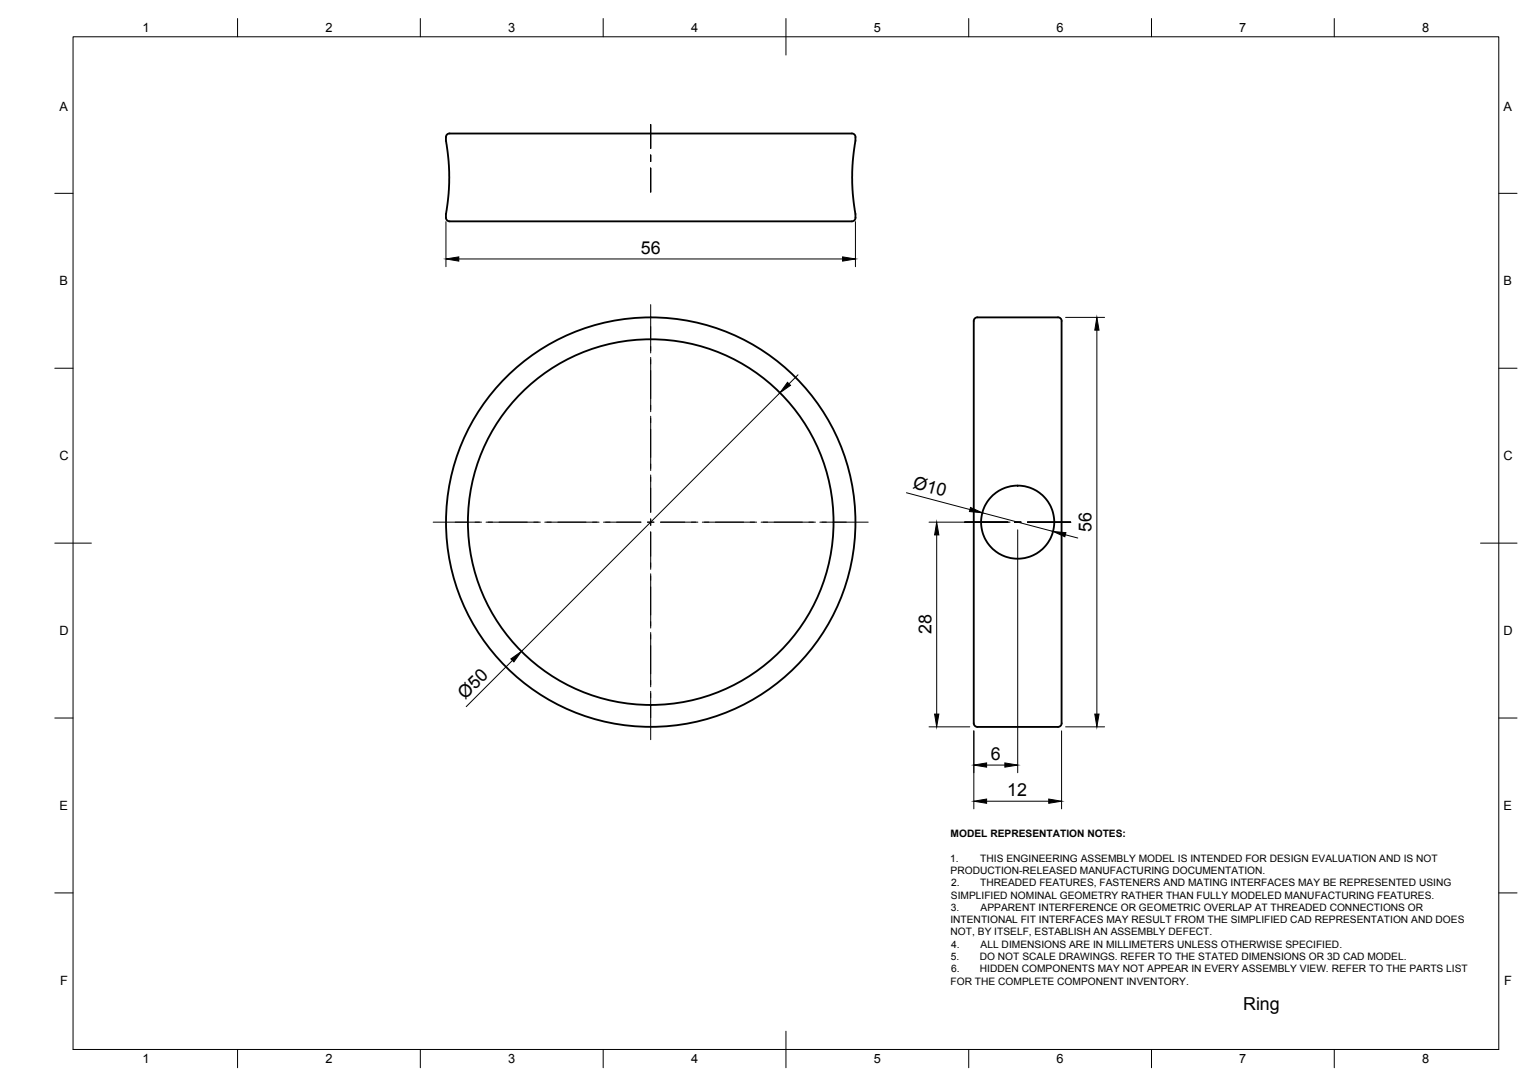
ISO-10303-21;
HEADER;
/* Generated by software containing ST-Developer
 * from STEP Tools, Inc. (www.steptools.com) 
 */

FILE_DESCRIPTION(
/* description */ (''),
/* implementation_level */ '2;1');

FILE_NAME(
/* name */ 'Ring.step',
/* time_stamp */ '2026-10-06T12:52:28-07:00',
/* author */ (''),
/* organization */ (''),
/* preprocessor_version */ 'ST-DEVELOPER v20.2',
/* originating_system */ 'Autodesk Translation Framework v15.15.0.0',
/* authorisation */ '');

FILE_SCHEMA (('AUTOMOTIVE_DESIGN { 1 0 10303 214 3 1 1 }'));
ENDSEC;

DATA;
#10=MECHANICAL_DESIGN_GEOMETRIC_PRESENTATION_REPRESENTATION('',(#73),#34403);
#57=SHAPE_REPRESENTATION_RELATIONSHIP('SRR','None',#34435,#65);
#65=ADVANCED_BREP_SHAPE_REPRESENTATION('',(#81),#34395);
#73=STYLED_ITEM('',(#34484),#81);
#81=MANIFOLD_SOLID_BREP('Body1',#4382);
#89=FACE_BOUND('',#751,.T.);
#90=FACE_BOUND('',#753,.T.);
#91=FACE_BOUND('',#754,.T.);
#92=FACE_BOUND('',#757,.T.);
#93=FACE_BOUND('',#758,.T.);
#94=FACE_BOUND('',#761,.T.);
#125=PLANE('',#4488);
#126=PLANE('',#4503);
#160=CIRCLE('',#4484,25.5);
#161=CIRCLE('',#4485,0.5);
#162=CIRCLE('',#4486,25.);
#163=CIRCLE('',#4487,25.);
#164=CIRCLE('',#4489,27.5);
#165=CIRCLE('',#4491,25.);
#166=CIRCLE('',#4492,25.);
#167=CIRCLE('',#4494,0.5);
#168=CIRCLE('',#4495,28.);
#169=CIRCLE('',#4496,28.);
#170=CIRCLE('',#4498,28.);
#171=CIRCLE('',#4499,28.);
#172=CIRCLE('',#4501,27.5);
#173=CIRCLE('',#4502,0.5);
#174=CIRCLE('',#4504,25.5);
#175=CIRCLE('',#4506,0.5);
#446=TOROIDAL_SURFACE('',#4483,25.5,0.5);
#447=TOROIDAL_SURFACE('',#4493,27.5,0.5);
#448=TOROIDAL_SURFACE('',#4500,27.5,0.5);
#449=TOROIDAL_SURFACE('',#4505,25.5,0.5);
#516=FACE_OUTER_BOUND('',#747,.T.);
#517=FACE_OUTER_BOUND('',#748,.T.);
#518=FACE_OUTER_BOUND('',#749,.T.);
#519=FACE_OUTER_BOUND('',#750,.T.);
#520=FACE_OUTER_BOUND('',#752,.T.);
#521=FACE_OUTER_BOUND('',#755,.T.);
#522=FACE_OUTER_BOUND('',#756,.T.);
#523=FACE_OUTER_BOUND('',#759,.T.);
#524=FACE_OUTER_BOUND('',#760,.T.);
#525=FACE_OUTER_BOUND('',#762,.T.);
#747=EDGE_LOOP('',(#2683,#2684,#2685,#2686,#2687,#2688));
#748=EDGE_LOOP('',(#2689,#2690,#2691,#2692,#2693,#2694));
#749=EDGE_LOOP('',(#2695,#2696,#2697,#2698,#2699));
#750=EDGE_LOOP('',(#2700));
#751=EDGE_LOOP('',(#2701));
#752=EDGE_LOOP('',(#2702,#2703,#2704,#2705,#2706,#2707));
#753=EDGE_LOOP('',(#2708,#2709));
#754=EDGE_LOOP('',(#2710,#2711));
#755=EDGE_LOOP('',(#2712,#2713,#2714,#2715,#2716));
#756=EDGE_LOOP('',(#2717,#2718,#2719,#2720,#2721,#2722));
#757=EDGE_LOOP('',(#2723,#2724));
#758=EDGE_LOOP('',(#2725,#2726));
#759=EDGE_LOOP('',(#2727,#2728,#2729,#2730,#2731));
#760=EDGE_LOOP('',(#2732));
#761=EDGE_LOOP('',(#2733));
#762=EDGE_LOOP('',(#2734,#2735,#2736,#2737,#2738));
#1014=LINE('',#6230,#1151);
#1015=LINE('',#6308,#1152);
#1016=LINE('',#6362,#1153);
#1017=LINE('',#6371,#1154);
#1151=VECTOR('',#5009,5.);
#1152=VECTOR('',#5012,5.);
#1153=VECTOR('',#5033,25.);
#1154=VECTOR('',#5044,28.);
#1288=B_SPLINE_CURVE_WITH_KNOTS('',3,(#6193,#6194,#6195,#6196,#6197,#6198,
#6199,#6200,#6201,#6202,#6203,#6204,#6205,#6206,#6207,#6208,#6209,#6210),
 .UNSPECIFIED.,.F.,.F.,(4,2,2,2,2,2,2,2,4),(0.,0.188782577961406,0.377565155922812,
0.566341063168598,0.755116970414385,0.94389287766017,1.13266878490596,1.32145136286736,
1.51023394082877),.UNSPECIFIED.);
#1289=B_SPLINE_CURVE_WITH_KNOTS('',3,(#6211,#6212,#6213,#6214,#6215,#6216,
#6217,#6218,#6219,#6220,#6221,#6222,#6223,#6224,#6225,#6226,#6227,#6228),
 .UNSPECIFIED.,.F.,.F.,(4,2,2,2,2,2,2,2,4),(1.51023394082877,1.69901651879018,
1.88779909675158,2.07657500399737,2.26535091124315,2.45412681848894,2.64290272573473,
2.83168530369613,3.02046788165754),.UNSPECIFIED.);
#1290=B_SPLINE_CURVE_WITH_KNOTS('',3,(#6232,#6233,#6234,#6235,#6236,#6237,
#6238,#6239,#6240,#6241,#6242,#6243,#6244,#6245,#6246,#6247,#6248,#6249),
 .UNSPECIFIED.,.F.,.F.,(4,2,2,2,2,2,2,2,4),(-3.02227736861757,-2.83337974067247,
-2.64448211272738,-2.45559506959528,-2.26670802646318,-2.07782098333108,
-1.88893394019898,-1.70003631225388,-1.51113868430879),.UNSPECIFIED.);
#1291=B_SPLINE_CURVE_WITH_KNOTS('',3,(#6250,#6251,#6252,#6253,#6254,#6255,
#6256,#6257,#6258,#6259,#6260,#6261,#6262,#6263,#6264,#6265,#6266,#6267),
 .UNSPECIFIED.,.F.,.F.,(4,2,2,2,2,2,2,2,4),(-1.51113868430879,-1.32224105636369,
-1.13334342841859,-0.944456385286492,-0.755569342154393,-0.566682299022294,
-0.377795255890194,-0.188897627945097,0.),.UNSPECIFIED.);
#1292=B_SPLINE_CURVE_WITH_KNOTS('',3,(#6271,#6272,#6273,#6274,#6275,#6276,
#6277,#6278,#6279,#6280,#6281,#6282,#6283,#6284,#6285,#6286,#6287,#6288),
 .UNSPECIFIED.,.F.,.F.,(4,2,2,2,2,2,2,2,4),(-3.02227736861757,-2.83337974067247,
-2.64448211272738,-2.45559506959528,-2.26670802646318,-2.07782098333108,
-1.88893394019898,-1.70003631225388,-1.51113868430879),.UNSPECIFIED.);
#1293=B_SPLINE_CURVE_WITH_KNOTS('',3,(#6289,#6290,#6291,#6292,#6293,#6294,
#6295,#6296,#6297,#6298,#6299,#6300,#6301,#6302,#6303,#6304,#6305,#6306),
 .UNSPECIFIED.,.F.,.F.,(4,2,2,2,2,2,2,2,4),(-1.51113868430879,-1.32224105636369,
-1.13334342841859,-0.944456385286492,-0.755569342154393,-0.566682299022294,
-0.377795255890194,-0.188897627945097,0.),.UNSPECIFIED.);
#1294=B_SPLINE_CURVE_WITH_KNOTS('',3,(#6310,#6311,#6312,#6313,#6314,#6315,
#6316,#6317,#6318,#6319,#6320,#6321,#6322,#6323,#6324,#6325,#6326,#6327),
 .UNSPECIFIED.,.F.,.F.,(4,2,2,2,2,2,2,2,4),(0.,0.188782577961406,0.377565155922812,
0.566341063168599,0.755116970414385,0.943892877660171,1.13266878490596,
1.32145136286736,1.51023394082877),.UNSPECIFIED.);
#1295=B_SPLINE_CURVE_WITH_KNOTS('',3,(#6328,#6329,#6330,#6331,#6332,#6333,
#6334,#6335,#6336,#6337,#6338,#6339,#6340,#6341,#6342,#6343,#6344,#6345),
 .UNSPECIFIED.,.F.,.F.,(4,2,2,2,2,2,2,2,4),(1.51023394082877,1.69901651879018,
1.88779909675158,2.07657500399737,2.26535091124315,2.45412681848894,2.64290272573473,
2.83168530369613,3.02046788165754),.UNSPECIFIED.);
#1540=VERTEX_POINT('',#6191);
#1541=VERTEX_POINT('',#6192);
#1542=VERTEX_POINT('',#6229);
#1543=VERTEX_POINT('',#6231);
#1544=VERTEX_POINT('',#6269);
#1545=VERTEX_POINT('',#6270);
#1546=VERTEX_POINT('',#6307);
#1547=VERTEX_POINT('',#6309);
#1548=VERTEX_POINT('',#6347);
#1549=VERTEX_POINT('',#6349);
#1550=VERTEX_POINT('',#6351);
#1551=VERTEX_POINT('',#6355);
#1552=VERTEX_POINT('',#6358);
#1553=VERTEX_POINT('',#6359);
#1554=VERTEX_POINT('',#6364);
#1555=VERTEX_POINT('',#6366);
#1556=VERTEX_POINT('',#6370);
#1557=VERTEX_POINT('',#6372);
#1558=VERTEX_POINT('',#6376);
#1559=VERTEX_POINT('',#6380);
#2006=EDGE_CURVE('',#1540,#1541,#1288,.T.);
#2007=EDGE_CURVE('',#1541,#1540,#1289,.T.);
#2008=EDGE_CURVE('',#1541,#1542,#1014,.T.);
#2009=EDGE_CURVE('',#1543,#1542,#1290,.T.);
#2010=EDGE_CURVE('',#1542,#1543,#1291,.T.);
#2011=EDGE_CURVE('',#1544,#1545,#1292,.T.);
#2012=EDGE_CURVE('',#1545,#1544,#1293,.T.);
#2013=EDGE_CURVE('',#1545,#1546,#1015,.T.);
#2014=EDGE_CURVE('',#1547,#1546,#1294,.T.);
#2015=EDGE_CURVE('',#1546,#1547,#1295,.T.);
#2016=EDGE_CURVE('',#1548,#1548,#160,.T.);
#2017=EDGE_CURVE('',#1548,#1549,#161,.T.);
#2018=EDGE_CURVE('',#1549,#1550,#162,.T.);
#2019=EDGE_CURVE('',#1550,#1549,#163,.T.);
#2020=EDGE_CURVE('',#1551,#1551,#164,.T.);
#2021=EDGE_CURVE('',#1552,#1553,#165,.T.);
#2022=EDGE_CURVE('',#1553,#1552,#166,.T.);
#2023=EDGE_CURVE('',#1553,#1550,#1016,.T.);
#2024=EDGE_CURVE('',#1551,#1554,#167,.T.);
#2025=EDGE_CURVE('',#1554,#1555,#168,.T.);
#2026=EDGE_CURVE('',#1555,#1554,#169,.T.);
#2027=EDGE_CURVE('',#1555,#1556,#1017,.T.);
#2028=EDGE_CURVE('',#1557,#1556,#170,.T.);
#2029=EDGE_CURVE('',#1556,#1557,#171,.T.);
#2030=EDGE_CURVE('',#1558,#1558,#172,.T.);
#2031=EDGE_CURVE('',#1558,#1557,#173,.T.);
#2032=EDGE_CURVE('',#1559,#1559,#174,.T.);
#2033=EDGE_CURVE('',#1559,#1552,#175,.T.);
#2683=ORIENTED_EDGE('',*,*,#2006,.F.);
#2684=ORIENTED_EDGE('',*,*,#2007,.F.);
#2685=ORIENTED_EDGE('',*,*,#2008,.T.);
#2686=ORIENTED_EDGE('',*,*,#2009,.F.);
#2687=ORIENTED_EDGE('',*,*,#2010,.F.);
#2688=ORIENTED_EDGE('',*,*,#2008,.F.);
#2689=ORIENTED_EDGE('',*,*,#2011,.F.);
#2690=ORIENTED_EDGE('',*,*,#2012,.F.);
#2691=ORIENTED_EDGE('',*,*,#2013,.T.);
#2692=ORIENTED_EDGE('',*,*,#2014,.F.);
#2693=ORIENTED_EDGE('',*,*,#2015,.F.);
#2694=ORIENTED_EDGE('',*,*,#2013,.F.);
#2695=ORIENTED_EDGE('',*,*,#2016,.T.);
#2696=ORIENTED_EDGE('',*,*,#2017,.T.);
#2697=ORIENTED_EDGE('',*,*,#2018,.T.);
#2698=ORIENTED_EDGE('',*,*,#2019,.T.);
#2699=ORIENTED_EDGE('',*,*,#2017,.F.);
#2700=ORIENTED_EDGE('',*,*,#2020,.F.);
#2701=ORIENTED_EDGE('',*,*,#2016,.F.);
#2702=ORIENTED_EDGE('',*,*,#2021,.F.);
#2703=ORIENTED_EDGE('',*,*,#2022,.F.);
#2704=ORIENTED_EDGE('',*,*,#2023,.T.);
#2705=ORIENTED_EDGE('',*,*,#2018,.F.);
#2706=ORIENTED_EDGE('',*,*,#2019,.F.);
#2707=ORIENTED_EDGE('',*,*,#2023,.F.);
#2708=ORIENTED_EDGE('',*,*,#2011,.T.);
#2709=ORIENTED_EDGE('',*,*,#2012,.T.);
#2710=ORIENTED_EDGE('',*,*,#2009,.T.);
#2711=ORIENTED_EDGE('',*,*,#2010,.T.);
#2712=ORIENTED_EDGE('',*,*,#2020,.T.);
#2713=ORIENTED_EDGE('',*,*,#2024,.T.);
#2714=ORIENTED_EDGE('',*,*,#2025,.T.);
#2715=ORIENTED_EDGE('',*,*,#2026,.T.);
#2716=ORIENTED_EDGE('',*,*,#2024,.F.);
#2717=ORIENTED_EDGE('',*,*,#2026,.F.);
#2718=ORIENTED_EDGE('',*,*,#2027,.T.);
#2719=ORIENTED_EDGE('',*,*,#2028,.F.);
#2720=ORIENTED_EDGE('',*,*,#2029,.F.);
#2721=ORIENTED_EDGE('',*,*,#2027,.F.);
#2722=ORIENTED_EDGE('',*,*,#2025,.F.);
#2723=ORIENTED_EDGE('',*,*,#2014,.T.);
#2724=ORIENTED_EDGE('',*,*,#2015,.T.);
#2725=ORIENTED_EDGE('',*,*,#2006,.T.);
#2726=ORIENTED_EDGE('',*,*,#2007,.T.);
#2727=ORIENTED_EDGE('',*,*,#2030,.T.);
#2728=ORIENTED_EDGE('',*,*,#2031,.T.);
#2729=ORIENTED_EDGE('',*,*,#2028,.T.);
#2730=ORIENTED_EDGE('',*,*,#2029,.T.);
#2731=ORIENTED_EDGE('',*,*,#2031,.F.);
#2732=ORIENTED_EDGE('',*,*,#2030,.F.);
#2733=ORIENTED_EDGE('',*,*,#2032,.F.);
#2734=ORIENTED_EDGE('',*,*,#2032,.T.);
#2735=ORIENTED_EDGE('',*,*,#2033,.T.);
#2736=ORIENTED_EDGE('',*,*,#2021,.T.);
#2737=ORIENTED_EDGE('',*,*,#2022,.T.);
#2738=ORIENTED_EDGE('',*,*,#2033,.F.);
#4037=CYLINDRICAL_SURFACE('',#4481,5.);
#4038=CYLINDRICAL_SURFACE('',#4482,5.);
#4039=CYLINDRICAL_SURFACE('',#4490,25.);
#4040=CYLINDRICAL_SURFACE('',#4497,28.);
#4151=ADVANCED_FACE('',(#516),#4037,.F.);
#4152=ADVANCED_FACE('',(#517),#4038,.F.);
#4153=ADVANCED_FACE('',(#518),#446,.T.);
#4154=ADVANCED_FACE('',(#519,#89),#125,.T.);
#4155=ADVANCED_FACE('',(#520,#90,#91),#4039,.F.);
#4156=ADVANCED_FACE('',(#521),#447,.T.);
#4157=ADVANCED_FACE('',(#522,#92,#93),#4040,.T.);
#4158=ADVANCED_FACE('',(#523),#448,.T.);
#4159=ADVANCED_FACE('',(#524,#94),#126,.F.);
#4160=ADVANCED_FACE('',(#525),#449,.T.);
#4382=CLOSED_SHELL('',(#4151,#4152,#4153,#4154,#4155,#4156,#4157,#4158,
#4159,#4160));
#4480=AXIS2_PLACEMENT_3D('',#6189,#5005,#5006);
#4481=AXIS2_PLACEMENT_3D('',#6190,#5007,#5008);
#4482=AXIS2_PLACEMENT_3D('',#6268,#5010,#5011);
#4483=AXIS2_PLACEMENT_3D('',#6346,#5013,#5014);
#4484=AXIS2_PLACEMENT_3D('',#6348,#5015,#5016);
#4485=AXIS2_PLACEMENT_3D('',#6350,#5017,#5018);
#4486=AXIS2_PLACEMENT_3D('',#6352,#5019,#5020);
#4487=AXIS2_PLACEMENT_3D('',#6353,#5021,#5022);
#4488=AXIS2_PLACEMENT_3D('',#6354,#5023,#5024);
#4489=AXIS2_PLACEMENT_3D('',#6356,#5025,#5026);
#4490=AXIS2_PLACEMENT_3D('',#6357,#5027,#5028);
#4491=AXIS2_PLACEMENT_3D('',#6360,#5029,#5030);
#4492=AXIS2_PLACEMENT_3D('',#6361,#5031,#5032);
#4493=AXIS2_PLACEMENT_3D('',#6363,#5034,#5035);
#4494=AXIS2_PLACEMENT_3D('',#6365,#5036,#5037);
#4495=AXIS2_PLACEMENT_3D('',#6367,#5038,#5039);
#4496=AXIS2_PLACEMENT_3D('',#6368,#5040,#5041);
#4497=AXIS2_PLACEMENT_3D('',#6369,#5042,#5043);
#4498=AXIS2_PLACEMENT_3D('',#6373,#5045,#5046);
#4499=AXIS2_PLACEMENT_3D('',#6374,#5047,#5048);
#4500=AXIS2_PLACEMENT_3D('',#6375,#5049,#5050);
#4501=AXIS2_PLACEMENT_3D('',#6377,#5051,#5052);
#4502=AXIS2_PLACEMENT_3D('',#6378,#5053,#5054);
#4503=AXIS2_PLACEMENT_3D('',#6379,#5055,#5056);
#4504=AXIS2_PLACEMENT_3D('',#6381,#5057,#5058);
#4505=AXIS2_PLACEMENT_3D('',#6382,#5059,#5060);
#4506=AXIS2_PLACEMENT_3D('',#6383,#5061,#5062);
#5005=DIRECTION('axis',(0.,0.,1.));
#5006=DIRECTION('refdir',(1.,0.,0.));
#5007=DIRECTION('center_axis',(0.,0.,1.));
#5008=DIRECTION('ref_axis',(1.,0.,0.));
#5009=DIRECTION('',(0.,0.,1.));
#5010=DIRECTION('center_axis',(0.,0.,1.));
#5011=DIRECTION('ref_axis',(1.,0.,0.));
#5012=DIRECTION('',(0.,0.,1.));
#5013=DIRECTION('center_axis',(0.,-1.,0.));
#5014=DIRECTION('ref_axis',(0.,0.,-1.));
#5015=DIRECTION('center_axis',(0.,1.,0.));
#5016=DIRECTION('ref_axis',(1.,0.,0.));
#5017=DIRECTION('center_axis',(-1.,0.,-1.22464679914735E-16));
#5018=DIRECTION('ref_axis',(-1.22464679914735E-16,0.,1.));
#5019=DIRECTION('center_axis',(0.,-1.,0.));
#5020=DIRECTION('ref_axis',(1.,0.,0.));
#5021=DIRECTION('center_axis',(0.,-1.,0.));
#5022=DIRECTION('ref_axis',(1.,0.,0.));
#5023=DIRECTION('center_axis',(0.,1.,0.));
#5024=DIRECTION('ref_axis',(1.,0.,0.));
#5025=DIRECTION('center_axis',(0.,-1.,0.));
#5026=DIRECTION('ref_axis',(1.,0.,0.));
#5027=DIRECTION('center_axis',(0.,1.,0.));
#5028=DIRECTION('ref_axis',(1.,0.,0.));
#5029=DIRECTION('center_axis',(0.,1.,0.));
#5030=DIRECTION('ref_axis',(1.,0.,0.));
#5031=DIRECTION('center_axis',(0.,1.,0.));
#5032=DIRECTION('ref_axis',(1.,0.,0.));
#5033=DIRECTION('',(0.,1.,0.));
#5034=DIRECTION('center_axis',(0.,1.,0.));
#5035=DIRECTION('ref_axis',(0.,0.,1.));
#5036=DIRECTION('center_axis',(-1.,0.,1.22464679914735E-16));
#5037=DIRECTION('ref_axis',(-1.22464679914735E-16,0.,-1.));
#5038=DIRECTION('center_axis',(0.,1.,0.));
#5039=DIRECTION('ref_axis',(1.,0.,0.));
#5040=DIRECTION('center_axis',(0.,1.,0.));
#5041=DIRECTION('ref_axis',(1.,0.,0.));
#5042=DIRECTION('center_axis',(0.,1.,0.));
#5043=DIRECTION('ref_axis',(1.,0.,0.));
#5044=DIRECTION('',(0.,-1.,0.));
#5045=DIRECTION('center_axis',(0.,-1.,0.));
#5046=DIRECTION('ref_axis',(1.,0.,0.));
#5047=DIRECTION('center_axis',(0.,-1.,0.));
#5048=DIRECTION('ref_axis',(1.,0.,0.));
#5049=DIRECTION('center_axis',(0.,-1.,0.));
#5050=DIRECTION('ref_axis',(0.,0.,-1.));
#5051=DIRECTION('center_axis',(0.,1.,0.));
#5052=DIRECTION('ref_axis',(1.,0.,0.));
#5053=DIRECTION('center_axis',(-1.,0.,-1.22464679914735E-16));
#5054=DIRECTION('ref_axis',(-1.22464679914735E-16,0.,1.));
#5055=DIRECTION('center_axis',(0.,1.,0.));
#5056=DIRECTION('ref_axis',(1.,0.,0.));
#5057=DIRECTION('center_axis',(0.,-1.,0.));
#5058=DIRECTION('ref_axis',(1.,0.,0.));
#5059=DIRECTION('center_axis',(0.,1.,0.));
#5060=DIRECTION('ref_axis',(0.,0.,1.));
#5061=DIRECTION('center_axis',(-1.,0.,1.22464679914735E-16));
#5062=DIRECTION('ref_axis',(-1.22464679914735E-16,0.,-1.));
#6189=CARTESIAN_POINT('',(0.,0.,0.));
#6190=CARTESIAN_POINT('Origin',(0.,0.,0.));
#6191=CARTESIAN_POINT('',(5.,0.,-27.5499546279118));
#6192=CARTESIAN_POINT('',(-5.,-3.06161699786838E-16,-27.5499546279118));
#6193=CARTESIAN_POINT('Ctrl Pts',(5.,1.38777878078145E-16,-27.5499546279118));
#6194=CARTESIAN_POINT('Ctrl Pts',(5.,0.629275259871354,-27.5499546279118));
#6195=CARTESIAN_POINT('Ctrl Pts',(4.87396226264421,1.29954919562912,-27.5737468441049));
#6196=CARTESIAN_POINT('Ctrl Pts',(4.36328000904425,2.53103238085929,-27.6591541770631));
#6197=CARTESIAN_POINT('Ctrl Pts',(3.97870723422023,3.09236057764524,-27.7194782327905));
#6198=CARTESIAN_POINT('Ctrl Pts',(3.09237623737018,3.9786915744953,-27.832297423241));
#6199=CARTESIAN_POINT('Ctrl Pts',(2.53104134263485,4.3632766282051,-27.8921989820475));
#6200=CARTESIAN_POINT('Ctrl Pts',(1.29953505458189,4.87396779126795,-27.9766356618315));
#6201=CARTESIAN_POINT('Ctrl Pts',(0.62925302415262,5.,-28.));
#6202=CARTESIAN_POINT('Ctrl Pts',(-0.62925302415262,5.,-28.));
#6203=CARTESIAN_POINT('Ctrl Pts',(-1.29953505458189,4.87396779126795,-27.9766356618315));
#6204=CARTESIAN_POINT('Ctrl Pts',(-2.53104134263485,4.3632766282051,-27.8921989820475));
#6205=CARTESIAN_POINT('Ctrl Pts',(-3.09237623737018,3.9786915744953,-27.832297423241));
#6206=CARTESIAN_POINT('Ctrl Pts',(-3.97870723422023,3.09236057764524,-27.7194782327905));
#6207=CARTESIAN_POINT('Ctrl Pts',(-4.36328000904425,2.53103238085929,-27.6591541770631));
#6208=CARTESIAN_POINT('Ctrl Pts',(-4.87396226264421,1.29954919562912,-27.5737468441049));
#6209=CARTESIAN_POINT('Ctrl Pts',(-5.,0.629275259871354,-27.5499546279118));
#6210=CARTESIAN_POINT('Ctrl Pts',(-5.,-1.38777878078145E-16,-27.5499546279118));
#6211=CARTESIAN_POINT('Ctrl Pts',(-5.,0.,-27.5499546279118));
#6212=CARTESIAN_POINT('Ctrl Pts',(-5.,-0.629275259871354,-27.5499546279118));
#6213=CARTESIAN_POINT('Ctrl Pts',(-4.87396226264421,-1.29954919562912,-27.5737468441049));
#6214=CARTESIAN_POINT('Ctrl Pts',(-4.36328000904425,-2.53103238085929,-27.6591541770631));
#6215=CARTESIAN_POINT('Ctrl Pts',(-3.97870723422023,-3.09236057764524,-27.7194782327905));
#6216=CARTESIAN_POINT('Ctrl Pts',(-3.09237623737018,-3.9786915744953,-27.832297423241));
#6217=CARTESIAN_POINT('Ctrl Pts',(-2.53104134263485,-4.3632766282051,-27.8921989820475));
#6218=CARTESIAN_POINT('Ctrl Pts',(-1.29953505458189,-4.87396779126795,-27.9766356618315));
#6219=CARTESIAN_POINT('Ctrl Pts',(-0.629253024152621,-5.,-28.));
#6220=CARTESIAN_POINT('Ctrl Pts',(0.629253024152618,-5.,-28.));
#6221=CARTESIAN_POINT('Ctrl Pts',(1.29953505458189,-4.87396779126795,-27.9766356618315));
#6222=CARTESIAN_POINT('Ctrl Pts',(2.53104134263485,-4.3632766282051,-27.8921989820475));
#6223=CARTESIAN_POINT('Ctrl Pts',(3.09237623737018,-3.9786915744953,-27.832297423241));
#6224=CARTESIAN_POINT('Ctrl Pts',(3.97870723422023,-3.09236057764525,-27.7194782327905));
#6225=CARTESIAN_POINT('Ctrl Pts',(4.36328000904425,-2.5310323808593,-27.6591541770631));
#6226=CARTESIAN_POINT('Ctrl Pts',(4.87396226264421,-1.29954919562912,-27.5737468441049));
#6227=CARTESIAN_POINT('Ctrl Pts',(5.,-0.629275259871355,-27.5499546279118));
#6228=CARTESIAN_POINT('Ctrl Pts',(5.,0.,-27.5499546279118));
#6229=CARTESIAN_POINT('',(-5.,-6.12323399573677E-16,-24.4948974278318));
#6230=CARTESIAN_POINT('',(-5.,-6.12323399573677E-16,0.));
#6231=CARTESIAN_POINT('',(5.,1.38777878078145E-16,-24.4948974278318));
#6232=CARTESIAN_POINT('Ctrl Pts',(5.,0.,-24.4948974278318));
#6233=CARTESIAN_POINT('Ctrl Pts',(5.,-0.62965875981699,-24.4948974278318));
#6234=CARTESIAN_POINT('Ctrl Pts',(4.87381398124307,-1.30008888580946,-24.5216938309223));
#6235=CARTESIAN_POINT('Ctrl Pts',(4.36302708824191,-2.53146002515027,-24.6177075396385));
#6236=CARTESIAN_POINT('Ctrl Pts',(3.97851551096044,-3.09255230090503,-24.6854542550966));
#6237=CARTESIAN_POINT('Ctrl Pts',(3.09257712322547,-3.97849068864001,-24.8120168819159));
#6238=CARTESIAN_POINT('Ctrl Pts',(2.53147430598813,-4.36302170772379,-24.8791673575932));
#6239=CARTESIAN_POINT('Ctrl Pts',(1.30006653040932,-4.87382271117917,-24.9738094323541));
#6240=CARTESIAN_POINT('Ctrl Pts',(0.629623477106996,-5.,-25.));
#6241=CARTESIAN_POINT('Ctrl Pts',(-0.629623477106999,-5.,-25.));
#6242=CARTESIAN_POINT('Ctrl Pts',(-1.30006653040933,-4.87382271117917,-24.9738094323541));
#6243=CARTESIAN_POINT('Ctrl Pts',(-2.53147430598813,-4.36302170772379,-24.8791673575932));
#6244=CARTESIAN_POINT('Ctrl Pts',(-3.09257712322547,-3.97849068864001,-24.8120168819159));
#6245=CARTESIAN_POINT('Ctrl Pts',(-3.97851551096044,-3.09255230090503,-24.6854542550966));
#6246=CARTESIAN_POINT('Ctrl Pts',(-4.36302708824191,-2.53146002515027,-24.6177075396385));
#6247=CARTESIAN_POINT('Ctrl Pts',(-4.87381398124307,-1.30008888580945,-24.5216938309223));
#6248=CARTESIAN_POINT('Ctrl Pts',(-5.,-0.62965875981699,-24.4948974278318));
#6249=CARTESIAN_POINT('Ctrl Pts',(-5.,4.16333634234434E-16,-24.4948974278318));
#6250=CARTESIAN_POINT('Ctrl Pts',(-5.,1.38777878078145E-16,-24.4948974278318));
#6251=CARTESIAN_POINT('Ctrl Pts',(-5.,0.62965875981699,-24.4948974278318));
#6252=CARTESIAN_POINT('Ctrl Pts',(-4.87381398124307,1.30008888580945,-24.5216938309223));
#6253=CARTESIAN_POINT('Ctrl Pts',(-4.36302708824191,2.53146002515027,-24.6177075396385));
#6254=CARTESIAN_POINT('Ctrl Pts',(-3.97851551096044,3.09255230090503,-24.6854542550966));
#6255=CARTESIAN_POINT('Ctrl Pts',(-3.09257712322547,3.97849068864001,-24.8120168819159));
#6256=CARTESIAN_POINT('Ctrl Pts',(-2.53147430598813,4.36302170772379,-24.8791673575932));
#6257=CARTESIAN_POINT('Ctrl Pts',(-1.30006653040932,4.87382271117917,-24.9738094323541));
#6258=CARTESIAN_POINT('Ctrl Pts',(-0.629623477106998,5.,-25.));
#6259=CARTESIAN_POINT('Ctrl Pts',(0.629623477106998,5.,-25.));
#6260=CARTESIAN_POINT('Ctrl Pts',(1.30006653040932,4.87382271117917,-24.9738094323541));
#6261=CARTESIAN_POINT('Ctrl Pts',(2.53147430598813,4.36302170772379,-24.8791673575932));
#6262=CARTESIAN_POINT('Ctrl Pts',(3.09257712322547,3.97849068864001,-24.8120168819159));
#6263=CARTESIAN_POINT('Ctrl Pts',(3.97851551096044,3.09255230090503,-24.6854542550966));
#6264=CARTESIAN_POINT('Ctrl Pts',(4.36302708824191,2.53146002515027,-24.6177075396385));
#6265=CARTESIAN_POINT('Ctrl Pts',(4.87381398124307,1.30008888580945,-24.5216938309223));
#6266=CARTESIAN_POINT('Ctrl Pts',(5.,0.62965875981699,-24.4948974278318));
#6267=CARTESIAN_POINT('Ctrl Pts',(5.,-2.77555756156289E-16,-24.4948974278318));
#6268=CARTESIAN_POINT('Origin',(0.,0.,0.));
#6269=CARTESIAN_POINT('',(5.,1.38777878078145E-16,24.4948974278318));
#6270=CARTESIAN_POINT('',(-5.,-6.12323399573677E-16,24.4948974278318));
#6271=CARTESIAN_POINT('Ctrl Pts',(5.,0.,24.4948974278318));
#6272=CARTESIAN_POINT('Ctrl Pts',(5.,0.62965875981699,24.4948974278318));
#6273=CARTESIAN_POINT('Ctrl Pts',(4.87381398124307,1.30008888580945,24.5216938309223));
#6274=CARTESIAN_POINT('Ctrl Pts',(4.36302708824191,2.53146002515027,24.6177075396385));
#6275=CARTESIAN_POINT('Ctrl Pts',(3.97851551096044,3.09255230090503,24.6854542550966));
#6276=CARTESIAN_POINT('Ctrl Pts',(3.09257712322547,3.97849068864001,24.8120168819159));
#6277=CARTESIAN_POINT('Ctrl Pts',(2.53147430598813,4.36302170772379,24.8791673575932));
#6278=CARTESIAN_POINT('Ctrl Pts',(1.30006653040932,4.87382271117917,24.9738094323541));
#6279=CARTESIAN_POINT('Ctrl Pts',(0.629623477106997,5.,25.));
#6280=CARTESIAN_POINT('Ctrl Pts',(-0.629623477106997,5.,25.));
#6281=CARTESIAN_POINT('Ctrl Pts',(-1.30006653040932,4.87382271117917,24.9738094323541));
#6282=CARTESIAN_POINT('Ctrl Pts',(-2.53147430598813,4.36302170772379,24.8791673575932));
#6283=CARTESIAN_POINT('Ctrl Pts',(-3.09257712322547,3.97849068864001,24.8120168819159));
#6284=CARTESIAN_POINT('Ctrl Pts',(-3.97851551096044,3.09255230090503,24.6854542550966));
#6285=CARTESIAN_POINT('Ctrl Pts',(-4.36302708824191,2.53146002515027,24.6177075396385));
#6286=CARTESIAN_POINT('Ctrl Pts',(-4.87381398124307,1.30008888580945,24.5216938309223));
#6287=CARTESIAN_POINT('Ctrl Pts',(-5.,0.62965875981699,24.4948974278318));
#6288=CARTESIAN_POINT('Ctrl Pts',(-5.,0.,24.4948974278318));
#6289=CARTESIAN_POINT('Ctrl Pts',(-5.,1.38777878078145E-16,24.4948974278318));
#6290=CARTESIAN_POINT('Ctrl Pts',(-5.,-0.62965875981699,24.4948974278318));
#6291=CARTESIAN_POINT('Ctrl Pts',(-4.87381398124307,-1.30008888580945,24.5216938309223));
#6292=CARTESIAN_POINT('Ctrl Pts',(-4.36302708824191,-2.53146002515027,24.6177075396385));
#6293=CARTESIAN_POINT('Ctrl Pts',(-3.97851551096044,-3.09255230090503,24.6854542550966));
#6294=CARTESIAN_POINT('Ctrl Pts',(-3.09257712322547,-3.97849068864001,24.8120168819159));
#6295=CARTESIAN_POINT('Ctrl Pts',(-2.53147430598813,-4.36302170772379,24.8791673575932));
#6296=CARTESIAN_POINT('Ctrl Pts',(-1.30006653040932,-4.87382271117917,24.9738094323541));
#6297=CARTESIAN_POINT('Ctrl Pts',(-0.629623477106999,-5.,25.));
#6298=CARTESIAN_POINT('Ctrl Pts',(0.629623477106997,-5.,25.));
#6299=CARTESIAN_POINT('Ctrl Pts',(1.30006653040932,-4.87382271117917,24.9738094323541));
#6300=CARTESIAN_POINT('Ctrl Pts',(2.53147430598813,-4.36302170772379,24.8791673575932));
#6301=CARTESIAN_POINT('Ctrl Pts',(3.09257712322547,-3.97849068864001,24.8120168819159));
#6302=CARTESIAN_POINT('Ctrl Pts',(3.97851551096044,-3.09255230090503,24.6854542550966));
#6303=CARTESIAN_POINT('Ctrl Pts',(4.36302708824191,-2.53146002515027,24.6177075396385));
#6304=CARTESIAN_POINT('Ctrl Pts',(4.87381398124307,-1.30008888580946,24.5216938309223));
#6305=CARTESIAN_POINT('Ctrl Pts',(5.,-0.62965875981699,24.4948974278318));
#6306=CARTESIAN_POINT('Ctrl Pts',(5.,0.,24.4948974278318));
#6307=CARTESIAN_POINT('',(-5.,-1.67383821708694E-16,27.5499546279118));
#6308=CARTESIAN_POINT('',(-5.,-6.12323399573677E-16,0.));
#6309=CARTESIAN_POINT('',(5.,0.,27.5499546279118));
#6310=CARTESIAN_POINT('Ctrl Pts',(5.,1.38777878078145E-16,27.5499546279118));
#6311=CARTESIAN_POINT('Ctrl Pts',(5.,-0.629275259871354,27.5499546279118));
#6312=CARTESIAN_POINT('Ctrl Pts',(4.87396226264421,-1.29954919562912,27.5737468441049));
#6313=CARTESIAN_POINT('Ctrl Pts',(4.36328000904425,-2.53103238085929,27.6591541770631));
#6314=CARTESIAN_POINT('Ctrl Pts',(3.97870723422023,-3.09236057764524,27.7194782327905));
#6315=CARTESIAN_POINT('Ctrl Pts',(3.09237623737018,-3.9786915744953,27.832297423241));
#6316=CARTESIAN_POINT('Ctrl Pts',(2.53104134263485,-4.3632766282051,27.8921989820475));
#6317=CARTESIAN_POINT('Ctrl Pts',(1.29953505458189,-4.87396779126795,27.9766356618315));
#6318=CARTESIAN_POINT('Ctrl Pts',(0.629253024152619,-5.,28.));
#6319=CARTESIAN_POINT('Ctrl Pts',(-0.629253024152621,-5.,28.));
#6320=CARTESIAN_POINT('Ctrl Pts',(-1.29953505458189,-4.87396779126795,27.9766356618315));
#6321=CARTESIAN_POINT('Ctrl Pts',(-2.53104134263485,-4.3632766282051,27.8921989820475));
#6322=CARTESIAN_POINT('Ctrl Pts',(-3.09237623737018,-3.9786915744953,27.832297423241));
#6323=CARTESIAN_POINT('Ctrl Pts',(-3.97870723422023,-3.09236057764524,27.7194782327905));
#6324=CARTESIAN_POINT('Ctrl Pts',(-4.36328000904426,-2.53103238085929,27.6591541770631));
#6325=CARTESIAN_POINT('Ctrl Pts',(-4.87396226264421,-1.29954919562912,27.5737468441049));
#6326=CARTESIAN_POINT('Ctrl Pts',(-5.,-0.629275259871353,27.5499546279118));
#6327=CARTESIAN_POINT('Ctrl Pts',(-5.,-1.38777878078145E-16,27.5499546279118));
#6328=CARTESIAN_POINT('Ctrl Pts',(-5.,2.77555756156289E-16,27.5499546279118));
#6329=CARTESIAN_POINT('Ctrl Pts',(-5.,0.629275259871354,27.5499546279118));
#6330=CARTESIAN_POINT('Ctrl Pts',(-4.87396226264421,1.29954919562912,27.5737468441049));
#6331=CARTESIAN_POINT('Ctrl Pts',(-4.36328000904425,2.53103238085929,27.6591541770631));
#6332=CARTESIAN_POINT('Ctrl Pts',(-3.97870723422023,3.09236057764524,27.7194782327905));
#6333=CARTESIAN_POINT('Ctrl Pts',(-3.09237623737018,3.9786915744953,27.832297423241));
#6334=CARTESIAN_POINT('Ctrl Pts',(-2.53104134263485,4.3632766282051,27.8921989820475));
#6335=CARTESIAN_POINT('Ctrl Pts',(-1.29953505458189,4.87396779126795,27.9766356618315));
#6336=CARTESIAN_POINT('Ctrl Pts',(-0.629253024152619,5.,28.));
#6337=CARTESIAN_POINT('Ctrl Pts',(0.629253024152621,5.,28.));
#6338=CARTESIAN_POINT('Ctrl Pts',(1.29953505458189,4.87396779126795,27.9766356618315));
#6339=CARTESIAN_POINT('Ctrl Pts',(2.53104134263485,4.3632766282051,27.8921989820475));
#6340=CARTESIAN_POINT('Ctrl Pts',(3.09237623737018,3.9786915744953,27.832297423241));
#6341=CARTESIAN_POINT('Ctrl Pts',(3.97870723422023,3.09236057764524,27.7194782327905));
#6342=CARTESIAN_POINT('Ctrl Pts',(4.36328000904425,2.53103238085929,27.6591541770631));
#6343=CARTESIAN_POINT('Ctrl Pts',(4.87396226264421,1.29954919562912,27.5737468441049));
#6344=CARTESIAN_POINT('Ctrl Pts',(5.,0.629275259871354,27.5499546279118));
#6345=CARTESIAN_POINT('Ctrl Pts',(5.,2.77555756156289E-16,27.5499546279118));
#6346=CARTESIAN_POINT('Origin',(0.,5.5,0.));
#6347=CARTESIAN_POINT('',(-3.12284933782575E-15,6.,25.5));
#6348=CARTESIAN_POINT('Origin',(0.,6.,0.));
#6349=CARTESIAN_POINT('',(-3.06161699786838E-15,5.5,25.));
#6350=CARTESIAN_POINT('Origin',(-3.12284933782575E-15,5.5,25.5));
#6351=CARTESIAN_POINT('',(-25.,5.5,-3.06161699786838E-15));
#6352=CARTESIAN_POINT('Origin',(0.,5.5,0.));
#6353=CARTESIAN_POINT('Origin',(0.,5.5,0.));
#6354=CARTESIAN_POINT('Origin',(0.,6.,0.));
#6355=CARTESIAN_POINT('',(-3.36777869765522E-15,6.,-27.5));
#6356=CARTESIAN_POINT('Origin',(0.,6.,0.));
#6357=CARTESIAN_POINT('Origin',(0.,0.,0.));
#6358=CARTESIAN_POINT('',(-3.06161699786838E-15,-5.5,-25.));
#6359=CARTESIAN_POINT('',(-25.,-5.5,3.06161699786838E-15));
#6360=CARTESIAN_POINT('Origin',(0.,-5.5,0.));
#6361=CARTESIAN_POINT('Origin',(0.,-5.5,0.));
#6362=CARTESIAN_POINT('',(-25.,0.,3.06161699786838E-15));
#6363=CARTESIAN_POINT('Origin',(0.,5.5,0.));
#6364=CARTESIAN_POINT('',(-3.42901103761259E-15,5.5,-28.));
#6365=CARTESIAN_POINT('Origin',(-3.36777869765522E-15,5.5,-27.5));
#6366=CARTESIAN_POINT('',(-28.,5.5,3.42901103761259E-15));
#6367=CARTESIAN_POINT('Origin',(0.,5.5,0.));
#6368=CARTESIAN_POINT('Origin',(0.,5.5,0.));
#6369=CARTESIAN_POINT('Origin',(0.,0.,0.));
#6370=CARTESIAN_POINT('',(-28.,-5.5,3.42901103761259E-15));
#6371=CARTESIAN_POINT('',(-28.,0.,3.42901103761259E-15));
#6372=CARTESIAN_POINT('',(-3.42901103761259E-15,-5.5,28.));
#6373=CARTESIAN_POINT('Origin',(0.,-5.5,0.));
#6374=CARTESIAN_POINT('Origin',(0.,-5.5,0.));
#6375=CARTESIAN_POINT('Origin',(0.,-5.5,0.));
#6376=CARTESIAN_POINT('',(-3.36777869765522E-15,-6.,27.5));
#6377=CARTESIAN_POINT('Origin',(0.,-6.,0.));
#6378=CARTESIAN_POINT('Origin',(-3.36777869765522E-15,-5.5,27.5));
#6379=CARTESIAN_POINT('Origin',(0.,-6.,0.));
#6380=CARTESIAN_POINT('',(-3.12284933782575E-15,-6.,-25.5));
#6381=CARTESIAN_POINT('Origin',(0.,-6.,0.));
#6382=CARTESIAN_POINT('Origin',(0.,-5.5,0.));
#6383=CARTESIAN_POINT('Origin',(-3.12284933782575E-15,-5.5,-25.5));
#34385=UNCERTAINTY_MEASURE_WITH_UNIT(LENGTH_MEASURE(0.01),#34404,
'DISTANCE_ACCURACY_VALUE',
'Maximum model space distance between geometric entities at asserted c
onnectivities');
#34393=UNCERTAINTY_MEASURE_WITH_UNIT(LENGTH_MEASURE(0.01),#34404,
'DISTANCE_ACCURACY_VALUE',
'Maximum model space distance between geometric entities at asserted c
onnectivities');
#34395=(
GEOMETRIC_REPRESENTATION_CONTEXT(3)
GLOBAL_UNCERTAINTY_ASSIGNED_CONTEXT((#34385))
GLOBAL_UNIT_ASSIGNED_CONTEXT((#34404,#34406,#34407))
REPRESENTATION_CONTEXT('','3D')
);
#34403=(
GEOMETRIC_REPRESENTATION_CONTEXT(3)
GLOBAL_UNCERTAINTY_ASSIGNED_CONTEXT((#34393))
GLOBAL_UNIT_ASSIGNED_CONTEXT((#34404,#34406,#34407))
REPRESENTATION_CONTEXT('','3D')
);
#34404=(
LENGTH_UNIT()
NAMED_UNIT(*)
SI_UNIT(.MILLI.,.METRE.)
);
#34406=(
NAMED_UNIT(*)
PLANE_ANGLE_UNIT()
SI_UNIT($,.RADIAN.)
);
#34407=(
NAMED_UNIT(*)
SI_UNIT($,.STERADIAN.)
SOLID_ANGLE_UNIT()
);
#34409=SHAPE_DEFINITION_REPRESENTATION(#34418,#34435);
#34418=PRODUCT_DEFINITION_SHAPE('',$,#34445);
#34435=SHAPE_REPRESENTATION('',(#4480),#34395);
#34443=PRODUCT_DEFINITION_CONTEXT('part definition',#34472,'design');
#34445=PRODUCT_DEFINITION('Ring','Ring',#34454,#34443);
#34454=PRODUCT_DEFINITION_FORMATION('',$,#34475);
#34472=APPLICATION_CONTEXT(
'Core Data for Automotive Mechanical Design Process');
#34473=PRODUCT_CONTEXT('part definition',#34472,'mechanical');
#34475=PRODUCT('Ring','Ring',$,(#34473));
#34484=PRESENTATION_STYLE_ASSIGNMENT((#34486));
#34486=SURFACE_STYLE_USAGE(.BOTH.,#34488);
#34488=SURFACE_SIDE_STYLE('',(#34490));
#34490=SURFACE_STYLE_FILL_AREA(#34492);
#34492=FILL_AREA_STYLE('Opaque(160,160,160)',(#34494));
#34494=FILL_AREA_STYLE_COLOUR('Opaque(160,160,160)',#34496);
#34496=COLOUR_RGB('Opaque(160,160,160)', 0.09019608, 0.27058824, 0.51372549);
ENDSEC;
END-ISO-10303-21;
